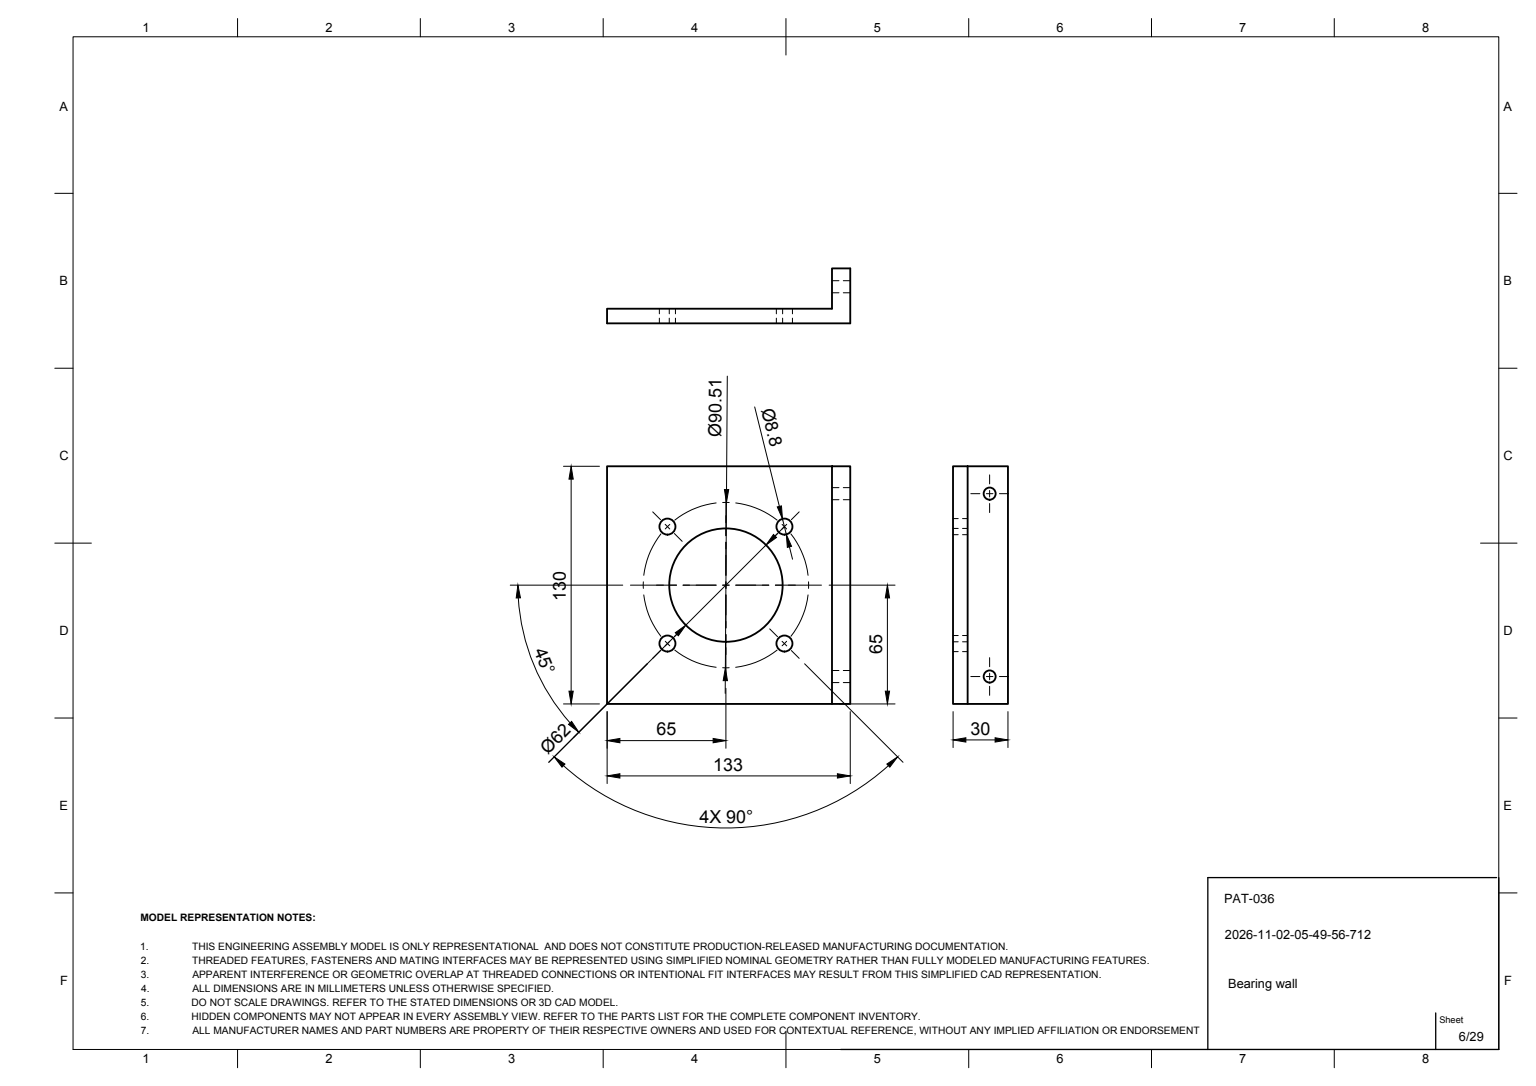
ISO-10303-21;
HEADER;
/* Generated by software containing ST-Developer
 * from STEP Tools, Inc. (www.steptools.com) 
 */

FILE_DESCRIPTION(
/* description */ ('Flange-mounted spindle'),
/* implementation_level */ '2;1');

FILE_NAME(
/* name */ 'Bearing wall.step',
/* time_stamp */ '2026-10-27T10:49:51-07:00',
/* author */ (''),
/* organization */ (''),
/* preprocessor_version */ 'ST-DEVELOPER v20.2',
/* originating_system */ 'Autodesk Translation Framework v15.17.0.0',
/* authorisation */ '');

FILE_SCHEMA (('AUTOMOTIVE_DESIGN { 1 0 10303 214 3 1 1 }'));
ENDSEC;

DATA;
#10=MECHANICAL_DESIGN_GEOMETRIC_PRESENTATION_REPRESENTATION('',(#339),#11764);
#285=SHAPE_REPRESENTATION_RELATIONSHIP('SRR','None',#11881,#312);
#312=ADVANCED_BREP_SHAPE_REPRESENTATION('',(#367),#11736);
#339=STYLED_ITEM('',(#12099),#367);
#367=MANIFOLD_SOLID_BREP('Body1',#6131);
#395=FACE_BOUND('',#1039,.T.);
#396=FACE_BOUND('',#1040,.T.);
#397=FACE_BOUND('',#1043,.T.);
#398=FACE_BOUND('',#1044,.T.);
#399=FACE_BOUND('',#1045,.T.);
#400=FACE_BOUND('',#1046,.T.);
#401=FACE_BOUND('',#1047,.T.);
#402=FACE_BOUND('',#1051,.T.);
#403=FACE_BOUND('',#1052,.T.);
#404=FACE_BOUND('',#1053,.T.);
#405=FACE_BOUND('',#1054,.T.);
#406=FACE_BOUND('',#1055,.T.);
#407=FACE_BOUND('',#1058,.T.);
#408=FACE_BOUND('',#1059,.T.);
#512=PLANE('',#6496);
#513=PLANE('',#6497);
#514=PLANE('',#6498);
#515=PLANE('',#6499);
#516=PLANE('',#6500);
#517=PLANE('',#6501);
#518=PLANE('',#6502);
#519=PLANE('',#6503);
#682=FACE_OUTER_BOUND('',#1031,.T.);
#683=FACE_OUTER_BOUND('',#1032,.T.);
#684=FACE_OUTER_BOUND('',#1033,.T.);
#685=FACE_OUTER_BOUND('',#1034,.T.);
#686=FACE_OUTER_BOUND('',#1035,.T.);
#687=FACE_OUTER_BOUND('',#1036,.T.);
#688=FACE_OUTER_BOUND('',#1037,.T.);
#689=FACE_OUTER_BOUND('',#1038,.T.);
#690=FACE_OUTER_BOUND('',#1041,.T.);
#691=FACE_OUTER_BOUND('',#1042,.T.);
#692=FACE_OUTER_BOUND('',#1048,.T.);
#693=FACE_OUTER_BOUND('',#1049,.T.);
#694=FACE_OUTER_BOUND('',#1050,.T.);
#695=FACE_OUTER_BOUND('',#1056,.T.);
#696=FACE_OUTER_BOUND('',#1057,.T.);
#1031=EDGE_LOOP('',(#4041,#4042,#4043,#4044));
#1032=EDGE_LOOP('',(#4045,#4046,#4047,#4048));
#1033=EDGE_LOOP('',(#4049,#4050,#4051,#4052));
#1034=EDGE_LOOP('',(#4053,#4054,#4055,#4056));
#1035=EDGE_LOOP('',(#4057,#4058,#4059,#4060));
#1036=EDGE_LOOP('',(#4061,#4062,#4063,#4064));
#1037=EDGE_LOOP('',(#4065,#4066,#4067,#4068));
#1038=EDGE_LOOP('',(#4069,#4070,#4071,#4072));
#1039=EDGE_LOOP('',(#4073));
#1040=EDGE_LOOP('',(#4074));
#1041=EDGE_LOOP('',(#4075,#4076,#4077,#4078));
#1042=EDGE_LOOP('',(#4079,#4080,#4081,#4082));
#1043=EDGE_LOOP('',(#4083));
#1044=EDGE_LOOP('',(#4084));
#1045=EDGE_LOOP('',(#4085));
#1046=EDGE_LOOP('',(#4086));
#1047=EDGE_LOOP('',(#4087));
#1048=EDGE_LOOP('',(#4088,#4089,#4090,#4091,#4092,#4093));
#1049=EDGE_LOOP('',(#4094,#4095,#4096,#4097,#4098,#4099));
#1050=EDGE_LOOP('',(#4100,#4101,#4102,#4103));
#1051=EDGE_LOOP('',(#4104));
#1052=EDGE_LOOP('',(#4105));
#1053=EDGE_LOOP('',(#4106));
#1054=EDGE_LOOP('',(#4107));
#1055=EDGE_LOOP('',(#4108));
#1056=EDGE_LOOP('',(#4109,#4110,#4111,#4112));
#1057=EDGE_LOOP('',(#4113,#4114,#4115,#4116));
#1058=EDGE_LOOP('',(#4117));
#1059=EDGE_LOOP('',(#4118));
#1493=LINE('',#9174,#1915);
#1494=LINE('',#9180,#1916);
#1495=LINE('',#9186,#1917);
#1496=LINE('',#9192,#1918);
#1497=LINE('',#9198,#1919);
#1498=LINE('',#9204,#1920);
#1499=LINE('',#9210,#1921);
#1500=LINE('',#9215,#1922);
#1501=LINE('',#9217,#1923);
#1502=LINE('',#9219,#1924);
#1503=LINE('',#9220,#1925);
#1504=LINE('',#9223,#1926);
#1505=LINE('',#9225,#1927);
#1506=LINE('',#9226,#1928);
#1507=LINE('',#9230,#1929);
#1508=LINE('',#9232,#1930);
#1509=LINE('',#9234,#1931);
#1510=LINE('',#9235,#1932);
#1511=LINE('',#9238,#1933);
#1512=LINE('',#9239,#1934);
#1513=LINE('',#9240,#1935);
#1514=LINE('',#9243,#1936);
#1515=LINE('',#9244,#1937);
#1516=LINE('',#9245,#1938);
#1517=LINE('',#9247,#1939);
#1915=VECTOR('',#7258,0.33);
#1916=VECTOR('',#7265,0.33);
#1917=VECTOR('',#7272,0.44);
#1918=VECTOR('',#7279,0.44);
#1919=VECTOR('',#7286,0.44);
#1920=VECTOR('',#7293,0.44);
#1921=VECTOR('',#7300,3.1);
#1922=VECTOR('',#7305,1.);
#1923=VECTOR('',#7306,1.);
#1924=VECTOR('',#7307,1.);
#1925=VECTOR('',#7308,1.);
#1926=VECTOR('',#7311,1.);
#1927=VECTOR('',#7312,1.);
#1928=VECTOR('',#7313,1.);
#1929=VECTOR('',#7316,1.);
#1930=VECTOR('',#7317,1.);
#1931=VECTOR('',#7318,1.);
#1932=VECTOR('',#7319,1.);
#1933=VECTOR('',#7322,1.);
#1934=VECTOR('',#7323,1.);
#1935=VECTOR('',#7324,1.);
#1936=VECTOR('',#7327,1.);
#1937=VECTOR('',#7328,1.);
#1938=VECTOR('',#7329,1.);
#1939=VECTOR('',#7332,1.);
#2327=CIRCLE('',#6476,0.33);
#2328=CIRCLE('',#6477,0.33);
#2329=CIRCLE('',#6479,0.33);
#2330=CIRCLE('',#6480,0.33);
#2331=CIRCLE('',#6482,0.44);
#2332=CIRCLE('',#6483,0.44);
#2333=CIRCLE('',#6485,0.44);
#2334=CIRCLE('',#6486,0.44);
#2335=CIRCLE('',#6488,0.44);
#2336=CIRCLE('',#6489,0.44);
#2337=CIRCLE('',#6491,0.44);
#2338=CIRCLE('',#6492,0.44);
#2339=CIRCLE('',#6494,3.1);
#2340=CIRCLE('',#6495,3.1);
#2661=VERTEX_POINT('',#9171);
#2662=VERTEX_POINT('',#9173);
#2663=VERTEX_POINT('',#9177);
#2664=VERTEX_POINT('',#9179);
#2665=VERTEX_POINT('',#9183);
#2666=VERTEX_POINT('',#9185);
#2667=VERTEX_POINT('',#9189);
#2668=VERTEX_POINT('',#9191);
#2669=VERTEX_POINT('',#9195);
#2670=VERTEX_POINT('',#9197);
#2671=VERTEX_POINT('',#9201);
#2672=VERTEX_POINT('',#9203);
#2673=VERTEX_POINT('',#9207);
#2674=VERTEX_POINT('',#9209);
#2675=VERTEX_POINT('',#9213);
#2676=VERTEX_POINT('',#9214);
#2677=VERTEX_POINT('',#9216);
#2678=VERTEX_POINT('',#9218);
#2679=VERTEX_POINT('',#9222);
#2680=VERTEX_POINT('',#9224);
#2681=VERTEX_POINT('',#9228);
#2682=VERTEX_POINT('',#9229);
#2683=VERTEX_POINT('',#9231);
#2684=VERTEX_POINT('',#9233);
#2685=VERTEX_POINT('',#9237);
#2686=VERTEX_POINT('',#9242);
#3213=EDGE_CURVE('',#2661,#2661,#2327,.T.);
#3214=EDGE_CURVE('',#2661,#2662,#1493,.T.);
#3215=EDGE_CURVE('',#2662,#2662,#2328,.T.);
#3216=EDGE_CURVE('',#2663,#2663,#2329,.T.);
#3217=EDGE_CURVE('',#2663,#2664,#1494,.T.);
#3218=EDGE_CURVE('',#2664,#2664,#2330,.T.);
#3219=EDGE_CURVE('',#2665,#2665,#2331,.T.);
#3220=EDGE_CURVE('',#2665,#2666,#1495,.T.);
#3221=EDGE_CURVE('',#2666,#2666,#2332,.T.);
#3222=EDGE_CURVE('',#2667,#2667,#2333,.T.);
#3223=EDGE_CURVE('',#2667,#2668,#1496,.T.);
#3224=EDGE_CURVE('',#2668,#2668,#2334,.T.);
#3225=EDGE_CURVE('',#2669,#2669,#2335,.T.);
#3226=EDGE_CURVE('',#2669,#2670,#1497,.T.);
#3227=EDGE_CURVE('',#2670,#2670,#2336,.T.);
#3228=EDGE_CURVE('',#2671,#2671,#2337,.T.);
#3229=EDGE_CURVE('',#2671,#2672,#1498,.T.);
#3230=EDGE_CURVE('',#2672,#2672,#2338,.T.);
#3231=EDGE_CURVE('',#2673,#2673,#2339,.T.);
#3232=EDGE_CURVE('',#2673,#2674,#1499,.T.);
#3233=EDGE_CURVE('',#2674,#2674,#2340,.T.);
#3234=EDGE_CURVE('',#2675,#2676,#1500,.T.);
#3235=EDGE_CURVE('',#2677,#2675,#1501,.T.);
#3236=EDGE_CURVE('',#2678,#2677,#1502,.T.);
#3237=EDGE_CURVE('',#2678,#2676,#1503,.T.);
#3238=EDGE_CURVE('',#2677,#2679,#1504,.T.);
#3239=EDGE_CURVE('',#2679,#2680,#1505,.T.);
#3240=EDGE_CURVE('',#2680,#2678,#1506,.T.);
#3241=EDGE_CURVE('',#2681,#2682,#1507,.T.);
#3242=EDGE_CURVE('',#2683,#2682,#1508,.T.);
#3243=EDGE_CURVE('',#2684,#2683,#1509,.T.);
#3244=EDGE_CURVE('',#2684,#2681,#1510,.T.);
#3245=EDGE_CURVE('',#2675,#2685,#1511,.T.);
#3246=EDGE_CURVE('',#2682,#2685,#1512,.T.);
#3247=EDGE_CURVE('',#2681,#2679,#1513,.T.);
#3248=EDGE_CURVE('',#2686,#2683,#1514,.T.);
#3249=EDGE_CURVE('',#2676,#2686,#1515,.T.);
#3250=EDGE_CURVE('',#2680,#2684,#1516,.T.);
#3251=EDGE_CURVE('',#2685,#2686,#1517,.T.);
#4041=ORIENTED_EDGE('',*,*,#3213,.F.);
#4042=ORIENTED_EDGE('',*,*,#3214,.T.);
#4043=ORIENTED_EDGE('',*,*,#3215,.F.);
#4044=ORIENTED_EDGE('',*,*,#3214,.F.);
#4045=ORIENTED_EDGE('',*,*,#3216,.F.);
#4046=ORIENTED_EDGE('',*,*,#3217,.T.);
#4047=ORIENTED_EDGE('',*,*,#3218,.F.);
#4048=ORIENTED_EDGE('',*,*,#3217,.F.);
#4049=ORIENTED_EDGE('',*,*,#3219,.F.);
#4050=ORIENTED_EDGE('',*,*,#3220,.T.);
#4051=ORIENTED_EDGE('',*,*,#3221,.F.);
#4052=ORIENTED_EDGE('',*,*,#3220,.F.);
#4053=ORIENTED_EDGE('',*,*,#3222,.F.);
#4054=ORIENTED_EDGE('',*,*,#3223,.T.);
#4055=ORIENTED_EDGE('',*,*,#3224,.F.);
#4056=ORIENTED_EDGE('',*,*,#3223,.F.);
#4057=ORIENTED_EDGE('',*,*,#3225,.F.);
#4058=ORIENTED_EDGE('',*,*,#3226,.T.);
#4059=ORIENTED_EDGE('',*,*,#3227,.F.);
#4060=ORIENTED_EDGE('',*,*,#3226,.F.);
#4061=ORIENTED_EDGE('',*,*,#3228,.F.);
#4062=ORIENTED_EDGE('',*,*,#3229,.T.);
#4063=ORIENTED_EDGE('',*,*,#3230,.F.);
#4064=ORIENTED_EDGE('',*,*,#3229,.F.);
#4065=ORIENTED_EDGE('',*,*,#3231,.F.);
#4066=ORIENTED_EDGE('',*,*,#3232,.T.);
#4067=ORIENTED_EDGE('',*,*,#3233,.F.);
#4068=ORIENTED_EDGE('',*,*,#3232,.F.);
#4069=ORIENTED_EDGE('',*,*,#3234,.F.);
#4070=ORIENTED_EDGE('',*,*,#3235,.F.);
#4071=ORIENTED_EDGE('',*,*,#3236,.F.);
#4072=ORIENTED_EDGE('',*,*,#3237,.T.);
#4073=ORIENTED_EDGE('',*,*,#3215,.T.);
#4074=ORIENTED_EDGE('',*,*,#3218,.T.);
#4075=ORIENTED_EDGE('',*,*,#3236,.T.);
#4076=ORIENTED_EDGE('',*,*,#3238,.T.);
#4077=ORIENTED_EDGE('',*,*,#3239,.T.);
#4078=ORIENTED_EDGE('',*,*,#3240,.T.);
#4079=ORIENTED_EDGE('',*,*,#3241,.T.);
#4080=ORIENTED_EDGE('',*,*,#3242,.F.);
#4081=ORIENTED_EDGE('',*,*,#3243,.F.);
#4082=ORIENTED_EDGE('',*,*,#3244,.T.);
#4083=ORIENTED_EDGE('',*,*,#3233,.T.);
#4084=ORIENTED_EDGE('',*,*,#3230,.T.);
#4085=ORIENTED_EDGE('',*,*,#3227,.T.);
#4086=ORIENTED_EDGE('',*,*,#3224,.T.);
#4087=ORIENTED_EDGE('',*,*,#3221,.T.);
#4088=ORIENTED_EDGE('',*,*,#3245,.T.);
#4089=ORIENTED_EDGE('',*,*,#3246,.F.);
#4090=ORIENTED_EDGE('',*,*,#3241,.F.);
#4091=ORIENTED_EDGE('',*,*,#3247,.T.);
#4092=ORIENTED_EDGE('',*,*,#3238,.F.);
#4093=ORIENTED_EDGE('',*,*,#3235,.T.);
#4094=ORIENTED_EDGE('',*,*,#3243,.T.);
#4095=ORIENTED_EDGE('',*,*,#3248,.F.);
#4096=ORIENTED_EDGE('',*,*,#3249,.F.);
#4097=ORIENTED_EDGE('',*,*,#3237,.F.);
#4098=ORIENTED_EDGE('',*,*,#3240,.F.);
#4099=ORIENTED_EDGE('',*,*,#3250,.T.);
#4100=ORIENTED_EDGE('',*,*,#3234,.T.);
#4101=ORIENTED_EDGE('',*,*,#3249,.T.);
#4102=ORIENTED_EDGE('',*,*,#3251,.F.);
#4103=ORIENTED_EDGE('',*,*,#3245,.F.);
#4104=ORIENTED_EDGE('',*,*,#3231,.T.);
#4105=ORIENTED_EDGE('',*,*,#3228,.T.);
#4106=ORIENTED_EDGE('',*,*,#3225,.T.);
#4107=ORIENTED_EDGE('',*,*,#3222,.T.);
#4108=ORIENTED_EDGE('',*,*,#3219,.T.);
#4109=ORIENTED_EDGE('',*,*,#3246,.T.);
#4110=ORIENTED_EDGE('',*,*,#3251,.T.);
#4111=ORIENTED_EDGE('',*,*,#3248,.T.);
#4112=ORIENTED_EDGE('',*,*,#3242,.T.);
#4113=ORIENTED_EDGE('',*,*,#3247,.F.);
#4114=ORIENTED_EDGE('',*,*,#3244,.F.);
#4115=ORIENTED_EDGE('',*,*,#3250,.F.);
#4116=ORIENTED_EDGE('',*,*,#3239,.F.);
#4117=ORIENTED_EDGE('',*,*,#3213,.T.);
#4118=ORIENTED_EDGE('',*,*,#3216,.T.);
#5627=CYLINDRICAL_SURFACE('',#6475,0.33);
#5628=CYLINDRICAL_SURFACE('',#6478,0.33);
#5629=CYLINDRICAL_SURFACE('',#6481,0.44);
#5630=CYLINDRICAL_SURFACE('',#6484,0.44);
#5631=CYLINDRICAL_SURFACE('',#6487,0.44);
#5632=CYLINDRICAL_SURFACE('',#6490,0.44);
#5633=CYLINDRICAL_SURFACE('',#6493,3.1);
#5793=ADVANCED_FACE('',(#682),#5627,.F.);
#5794=ADVANCED_FACE('',(#683),#5628,.F.);
#5795=ADVANCED_FACE('',(#684),#5629,.F.);
#5796=ADVANCED_FACE('',(#685),#5630,.F.);
#5797=ADVANCED_FACE('',(#686),#5631,.F.);
#5798=ADVANCED_FACE('',(#687),#5632,.F.);
#5799=ADVANCED_FACE('',(#688),#5633,.F.);
#5800=ADVANCED_FACE('',(#689,#395,#396),#512,.T.);
#5801=ADVANCED_FACE('',(#690),#513,.F.);
#5802=ADVANCED_FACE('',(#691,#397,#398,#399,#400,#401),#514,.T.);
#5803=ADVANCED_FACE('',(#692),#515,.T.);
#5804=ADVANCED_FACE('',(#693),#516,.T.);
#5805=ADVANCED_FACE('',(#694,#402,#403,#404,#405,#406),#517,.T.);
#5806=ADVANCED_FACE('',(#695),#518,.T.);
#5807=ADVANCED_FACE('',(#696,#407,#408),#519,.F.);
#6131=CLOSED_SHELL('',(#5793,#5794,#5795,#5796,#5797,#5798,#5799,#5800,
#5801,#5802,#5803,#5804,#5805,#5806,#5807));
#6474=AXIS2_PLACEMENT_3D('',#9169,#7252,#7253);
#6475=AXIS2_PLACEMENT_3D('',#9170,#7254,#7255);
#6476=AXIS2_PLACEMENT_3D('',#9172,#7256,#7257);
#6477=AXIS2_PLACEMENT_3D('',#9175,#7259,#7260);
#6478=AXIS2_PLACEMENT_3D('',#9176,#7261,#7262);
#6479=AXIS2_PLACEMENT_3D('',#9178,#7263,#7264);
#6480=AXIS2_PLACEMENT_3D('',#9181,#7266,#7267);
#6481=AXIS2_PLACEMENT_3D('',#9182,#7268,#7269);
#6482=AXIS2_PLACEMENT_3D('',#9184,#7270,#7271);
#6483=AXIS2_PLACEMENT_3D('',#9187,#7273,#7274);
#6484=AXIS2_PLACEMENT_3D('',#9188,#7275,#7276);
#6485=AXIS2_PLACEMENT_3D('',#9190,#7277,#7278);
#6486=AXIS2_PLACEMENT_3D('',#9193,#7280,#7281);
#6487=AXIS2_PLACEMENT_3D('',#9194,#7282,#7283);
#6488=AXIS2_PLACEMENT_3D('',#9196,#7284,#7285);
#6489=AXIS2_PLACEMENT_3D('',#9199,#7287,#7288);
#6490=AXIS2_PLACEMENT_3D('',#9200,#7289,#7290);
#6491=AXIS2_PLACEMENT_3D('',#9202,#7291,#7292);
#6492=AXIS2_PLACEMENT_3D('',#9205,#7294,#7295);
#6493=AXIS2_PLACEMENT_3D('',#9206,#7296,#7297);
#6494=AXIS2_PLACEMENT_3D('',#9208,#7298,#7299);
#6495=AXIS2_PLACEMENT_3D('',#9211,#7301,#7302);
#6496=AXIS2_PLACEMENT_3D('',#9212,#7303,#7304);
#6497=AXIS2_PLACEMENT_3D('',#9221,#7309,#7310);
#6498=AXIS2_PLACEMENT_3D('',#9227,#7314,#7315);
#6499=AXIS2_PLACEMENT_3D('',#9236,#7320,#7321);
#6500=AXIS2_PLACEMENT_3D('',#9241,#7325,#7326);
#6501=AXIS2_PLACEMENT_3D('',#9246,#7330,#7331);
#6502=AXIS2_PLACEMENT_3D('',#9248,#7333,#7334);
#6503=AXIS2_PLACEMENT_3D('',#9249,#7335,#7336);
#7252=DIRECTION('axis',(0.,0.,1.));
#7253=DIRECTION('refdir',(1.,0.,0.));
#7254=DIRECTION('center_axis',(0.,0.,1.));
#7255=DIRECTION('ref_axis',(1.,0.,0.));
#7256=DIRECTION('center_axis',(0.,0.,1.));
#7257=DIRECTION('ref_axis',(1.,0.,0.));
#7258=DIRECTION('',(0.,0.,1.));
#7259=DIRECTION('center_axis',(0.,0.,-1.));
#7260=DIRECTION('ref_axis',(1.,0.,0.));
#7261=DIRECTION('center_axis',(0.,0.,1.));
#7262=DIRECTION('ref_axis',(1.,0.,0.));
#7263=DIRECTION('center_axis',(0.,0.,1.));
#7264=DIRECTION('ref_axis',(1.,0.,0.));
#7265=DIRECTION('',(0.,0.,1.));
#7266=DIRECTION('center_axis',(0.,0.,-1.));
#7267=DIRECTION('ref_axis',(1.,0.,0.));
#7268=DIRECTION('center_axis',(0.,1.,0.));
#7269=DIRECTION('ref_axis',(1.,0.,0.));
#7270=DIRECTION('center_axis',(0.,1.,0.));
#7271=DIRECTION('ref_axis',(1.,0.,0.));
#7272=DIRECTION('',(0.,1.,0.));
#7273=DIRECTION('center_axis',(0.,-1.,0.));
#7274=DIRECTION('ref_axis',(1.,0.,0.));
#7275=DIRECTION('center_axis',(0.,1.,0.));
#7276=DIRECTION('ref_axis',(1.,0.,0.));
#7277=DIRECTION('center_axis',(0.,1.,0.));
#7278=DIRECTION('ref_axis',(1.,0.,0.));
#7279=DIRECTION('',(0.,1.,0.));
#7280=DIRECTION('center_axis',(0.,-1.,0.));
#7281=DIRECTION('ref_axis',(1.,0.,0.));
#7282=DIRECTION('center_axis',(0.,1.,0.));
#7283=DIRECTION('ref_axis',(1.,0.,0.));
#7284=DIRECTION('center_axis',(0.,1.,0.));
#7285=DIRECTION('ref_axis',(1.,0.,0.));
#7286=DIRECTION('',(0.,1.,0.));
#7287=DIRECTION('center_axis',(0.,-1.,0.));
#7288=DIRECTION('ref_axis',(1.,0.,0.));
#7289=DIRECTION('center_axis',(0.,1.,0.));
#7290=DIRECTION('ref_axis',(1.,0.,0.));
#7291=DIRECTION('center_axis',(0.,1.,0.));
#7292=DIRECTION('ref_axis',(1.,0.,0.));
#7293=DIRECTION('',(0.,1.,0.));
#7294=DIRECTION('center_axis',(0.,-1.,0.));
#7295=DIRECTION('ref_axis',(1.,0.,0.));
#7296=DIRECTION('center_axis',(0.,1.,0.));
#7297=DIRECTION('ref_axis',(1.,0.,0.));
#7298=DIRECTION('center_axis',(0.,1.,0.));
#7299=DIRECTION('ref_axis',(1.,0.,0.));
#7300=DIRECTION('',(0.,1.,0.));
#7301=DIRECTION('center_axis',(0.,-1.,0.));
#7302=DIRECTION('ref_axis',(1.,0.,0.));
#7303=DIRECTION('center_axis',(0.,0.,1.));
#7304=DIRECTION('ref_axis',(1.,0.,0.));
#7305=DIRECTION('',(1.,0.,0.));
#7306=DIRECTION('',(0.,1.,0.));
#7307=DIRECTION('',(-1.,0.,0.));
#7308=DIRECTION('',(0.,1.,0.));
#7309=DIRECTION('center_axis',(0.,1.,0.));
#7310=DIRECTION('ref_axis',(1.,0.,0.));
#7311=DIRECTION('',(0.,0.,-1.));
#7312=DIRECTION('',(1.,0.,0.));
#7313=DIRECTION('',(0.,0.,1.));
#7314=DIRECTION('center_axis',(0.,1.,0.));
#7315=DIRECTION('ref_axis',(-1.,0.,0.));
#7316=DIRECTION('',(0.,0.,1.));
#7317=DIRECTION('',(-1.,0.,0.));
#7318=DIRECTION('',(0.,0.,1.));
#7319=DIRECTION('',(-1.,0.,0.));
#7320=DIRECTION('center_axis',(-1.,0.,0.));
#7321=DIRECTION('ref_axis',(0.,-1.,0.));
#7322=DIRECTION('',(0.,0.,1.));
#7323=DIRECTION('',(0.,-1.,0.));
#7324=DIRECTION('',(0.,-1.,0.));
#7325=DIRECTION('center_axis',(1.,0.,0.));
#7326=DIRECTION('ref_axis',(0.,1.,0.));
#7327=DIRECTION('',(0.,1.,0.));
#7328=DIRECTION('',(0.,0.,1.));
#7329=DIRECTION('',(0.,1.,0.));
#7330=DIRECTION('center_axis',(0.,-1.,0.));
#7331=DIRECTION('ref_axis',(1.,0.,0.));
#7332=DIRECTION('',(1.,0.,0.));
#7333=DIRECTION('center_axis',(0.,0.,1.));
#7334=DIRECTION('ref_axis',(1.,0.,0.));
#7335=DIRECTION('center_axis',(0.,0.,1.));
#7336=DIRECTION('ref_axis',(1.,0.,0.));
#9169=CARTESIAN_POINT('',(0.,0.,0.));
#9170=CARTESIAN_POINT('Origin',(-5.,-2.5,1.1));
#9171=CARTESIAN_POINT('',(-5.33,-2.5,1.2));
#9172=CARTESIAN_POINT('Origin',(-5.,-2.5,1.2));
#9173=CARTESIAN_POINT('',(-5.33,-2.5,2.2));
#9174=CARTESIAN_POINT('',(-5.33,-2.5,1.1));
#9175=CARTESIAN_POINT('Origin',(-5.,-2.5,2.2));
#9176=CARTESIAN_POINT('Origin',(5.,-2.5,1.1));
#9177=CARTESIAN_POINT('',(4.67,-2.5,1.2));
#9178=CARTESIAN_POINT('Origin',(5.,-2.5,1.2));
#9179=CARTESIAN_POINT('',(4.67,-2.5,2.2));
#9180=CARTESIAN_POINT('',(4.67,-2.5,1.1));
#9181=CARTESIAN_POINT('Origin',(5.,-2.5,2.2));
#9182=CARTESIAN_POINT('Origin',(3.2,-1.4,4.8));
#9183=CARTESIAN_POINT('',(2.76,-1.3,4.8));
#9184=CARTESIAN_POINT('Origin',(3.2,-1.3,4.8));
#9185=CARTESIAN_POINT('',(2.76,-0.5,4.8));
#9186=CARTESIAN_POINT('',(2.76,-1.4,4.8));
#9187=CARTESIAN_POINT('Origin',(3.2,-0.5,4.8));
#9188=CARTESIAN_POINT('Origin',(-3.2,-1.4,11.2));
#9189=CARTESIAN_POINT('',(-3.64,-1.3,11.2));
#9190=CARTESIAN_POINT('Origin',(-3.2,-1.3,11.2));
#9191=CARTESIAN_POINT('',(-3.64,-0.5,11.2));
#9192=CARTESIAN_POINT('',(-3.64,-1.4,11.2));
#9193=CARTESIAN_POINT('Origin',(-3.2,-0.5,11.2));
#9194=CARTESIAN_POINT('Origin',(-3.2,-1.4,4.8));
#9195=CARTESIAN_POINT('',(-3.64,-1.3,4.8));
#9196=CARTESIAN_POINT('Origin',(-3.2,-1.3,4.8));
#9197=CARTESIAN_POINT('',(-3.64,-0.5,4.8));
#9198=CARTESIAN_POINT('',(-3.64,-1.4,4.8));
#9199=CARTESIAN_POINT('Origin',(-3.2,-0.5,4.8));
#9200=CARTESIAN_POINT('Origin',(3.2,-1.4,11.2));
#9201=CARTESIAN_POINT('',(2.76,-1.3,11.2));
#9202=CARTESIAN_POINT('Origin',(3.2,-1.3,11.2));
#9203=CARTESIAN_POINT('',(2.76,-0.5,11.2));
#9204=CARTESIAN_POINT('',(2.76,-1.4,11.2));
#9205=CARTESIAN_POINT('Origin',(3.2,-0.5,11.2));
#9206=CARTESIAN_POINT('Origin',(0.,-1.4,8.));
#9207=CARTESIAN_POINT('',(-3.1,-1.3,8.));
#9208=CARTESIAN_POINT('Origin',(0.,-1.3,8.));
#9209=CARTESIAN_POINT('',(-3.1,-0.5,8.));
#9210=CARTESIAN_POINT('',(-3.1,-1.4,8.));
#9211=CARTESIAN_POINT('Origin',(0.,-0.5,8.));
#9212=CARTESIAN_POINT('Origin',(-6.5,-3.5,2.2));
#9213=CARTESIAN_POINT('',(-6.5,-1.3,2.2));
#9214=CARTESIAN_POINT('',(6.5,-1.3,2.2));
#9215=CARTESIAN_POINT('',(-6.5,-1.3,2.2));
#9216=CARTESIAN_POINT('',(-6.5,-3.5,2.2));
#9217=CARTESIAN_POINT('',(-6.5,-3.5,2.2));
#9218=CARTESIAN_POINT('',(6.5,-3.5,2.2));
#9219=CARTESIAN_POINT('',(6.5,-3.5,2.2));
#9220=CARTESIAN_POINT('',(6.5,-3.5,2.2));
#9221=CARTESIAN_POINT('Origin',(0.,-3.5,1.7));
#9222=CARTESIAN_POINT('',(-6.5,-3.5,1.2));
#9223=CARTESIAN_POINT('',(-6.5,-3.5,2.2));
#9224=CARTESIAN_POINT('',(6.5,-3.5,1.2));
#9225=CARTESIAN_POINT('',(-6.5,-3.5,1.2));
#9226=CARTESIAN_POINT('',(6.5,-3.5,1.2));
#9227=CARTESIAN_POINT('Origin',(6.5,-0.5,1.2));
#9228=CARTESIAN_POINT('',(-6.5,-0.5,1.2));
#9229=CARTESIAN_POINT('',(-6.5,-0.5,14.5));
#9230=CARTESIAN_POINT('',(-6.5,-0.5,1.2));
#9231=CARTESIAN_POINT('',(6.5,-0.5,14.5));
#9232=CARTESIAN_POINT('',(6.5,-0.5,14.5));
#9233=CARTESIAN_POINT('',(6.5,-0.5,1.2));
#9234=CARTESIAN_POINT('',(6.5,-0.5,1.2));
#9235=CARTESIAN_POINT('',(6.5,-0.5,1.2));
#9236=CARTESIAN_POINT('Origin',(-6.5,-0.5,1.2));
#9237=CARTESIAN_POINT('',(-6.5,-1.3,14.5));
#9238=CARTESIAN_POINT('',(-6.5,-1.3,1.2));
#9239=CARTESIAN_POINT('',(-6.5,-0.5,14.5));
#9240=CARTESIAN_POINT('',(-6.5,-0.5,1.2));
#9241=CARTESIAN_POINT('Origin',(6.5,-1.3,1.2));
#9242=CARTESIAN_POINT('',(6.5,-1.3,14.5));
#9243=CARTESIAN_POINT('',(6.5,-1.3,14.5));
#9244=CARTESIAN_POINT('',(6.5,-1.3,1.2));
#9245=CARTESIAN_POINT('',(6.5,-3.5,1.2));
#9246=CARTESIAN_POINT('Origin',(-6.5,-1.3,1.2));
#9247=CARTESIAN_POINT('',(-6.5,-1.3,14.5));
#9248=CARTESIAN_POINT('Origin',(0.,-0.9,14.5));
#9249=CARTESIAN_POINT('Origin',(0.,-0.9,1.2));
#11704=UNCERTAINTY_MEASURE_WITH_UNIT(LENGTH_MEASURE(0.001),#11765,
'DISTANCE_ACCURACY_VALUE',
'Maximum model space distance between geometric entities at asserted c
onnectivities');
#11732=UNCERTAINTY_MEASURE_WITH_UNIT(LENGTH_MEASURE(0.001),#11765,
'DISTANCE_ACCURACY_VALUE',
'Maximum model space distance between geometric entities at asserted c
onnectivities');
#11736=(
GEOMETRIC_REPRESENTATION_CONTEXT(3)
GLOBAL_UNCERTAINTY_ASSIGNED_CONTEXT((#11704))
GLOBAL_UNIT_ASSIGNED_CONTEXT((#11765,#11767,#11768))
REPRESENTATION_CONTEXT('','3D')
);
#11764=(
GEOMETRIC_REPRESENTATION_CONTEXT(3)
GLOBAL_UNCERTAINTY_ASSIGNED_CONTEXT((#11732))
GLOBAL_UNIT_ASSIGNED_CONTEXT((#11765,#11767,#11768))
REPRESENTATION_CONTEXT('','3D')
);
#11765=(
LENGTH_UNIT()
NAMED_UNIT(*)
SI_UNIT(.CENTI.,.METRE.)
);
#11767=(
NAMED_UNIT(*)
PLANE_ANGLE_UNIT()
SI_UNIT($,.RADIAN.)
);
#11768=(
NAMED_UNIT(*)
SI_UNIT($,.STERADIAN.)
SOLID_ANGLE_UNIT()
);
#11772=SHAPE_DEFINITION_REPRESENTATION(#11803,#11881);
#11803=PRODUCT_DEFINITION_SHAPE('',$,#11913);
#11881=SHAPE_REPRESENTATION('',(#6474),#11736);
#11909=PRODUCT_DEFINITION_CONTEXT('part definition',#12004,'design');
#11913=PRODUCT_DEFINITION('Bearing wall','Bearing wall',#11944,#11909);
#11944=PRODUCT_DEFINITION_FORMATION('',$,#12009);
#12004=APPLICATION_CONTEXT(
'Core Data for Automotive Mechanical Design Process');
#12005=PRODUCT_CONTEXT('part definition',#12004,'mechanical');
#12009=PRODUCT('Bearing wall','Bearing wall','Bearing wall',(#12005));
#12093=COLOUR_RGB('Grey',0.48,0.52,0.57);
#12094=FILL_AREA_STYLE_COLOUR('',#12093);
#12095=FILL_AREA_STYLE('',(#12094));
#12096=SURFACE_STYLE_FILL_AREA(#12095);
#12097=SURFACE_SIDE_STYLE('',(#12096));
#12098=SURFACE_STYLE_USAGE(.BOTH.,#12097);
#12099=PRESENTATION_STYLE_ASSIGNMENT((#12098));
ENDSEC;
END-ISO-10303-21;
